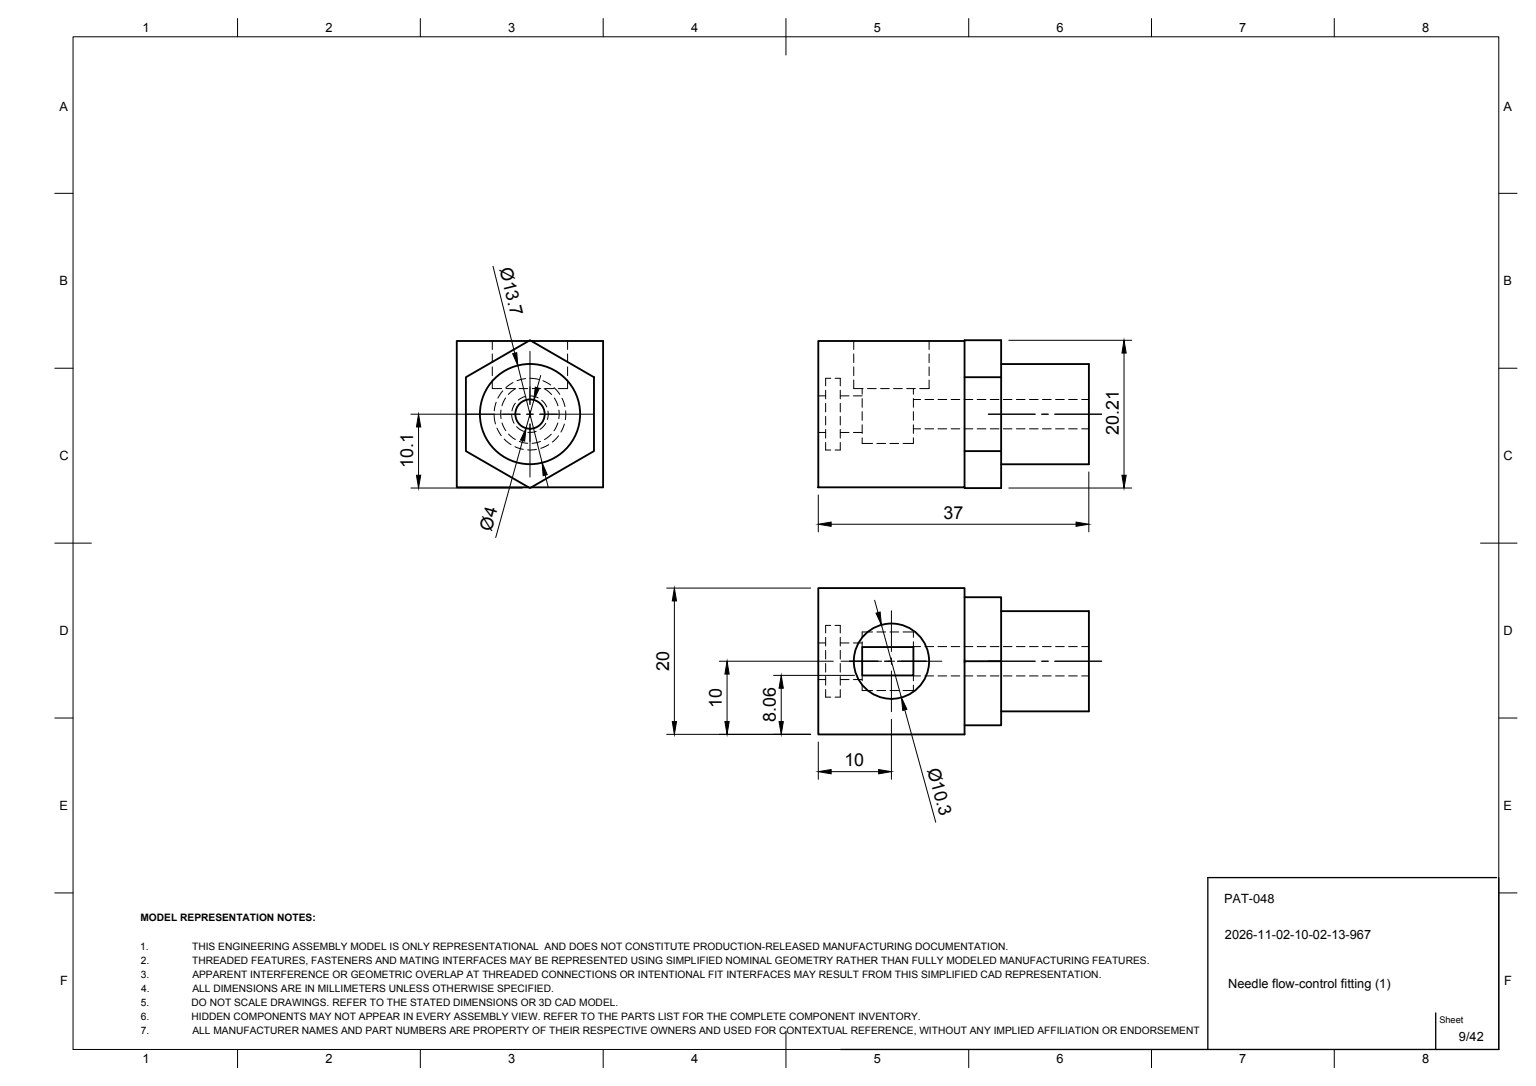
ISO-10303-21;
HEADER;
/* Generated by software containing ST-Developer
 * from STEP Tools, Inc. (www.steptools.com) 
 */

FILE_DESCRIPTION(
/* description */ ('Guided pneumatic stop gate'),
/* implementation_level */ '2;1');

FILE_NAME(
/* name */ 'Needle flow-control fitting (1).step',
/* time_stamp */ '2026-10-27T21:43:45-07:00',
/* author */ (''),
/* organization */ (''),
/* preprocessor_version */ 'ST-DEVELOPER v20.2',
/* originating_system */ 'Autodesk Translation Framework v15.17.0.0',
/* authorisation */ '');

FILE_SCHEMA (('AUTOMOTIVE_DESIGN { 1 0 10303 214 3 1 1 }'));
ENDSEC;

DATA;
#10=MECHANICAL_DESIGN_GEOMETRIC_PRESENTATION_REPRESENTATION('',(#539),#14392);
#455=SHAPE_REPRESENTATION_RELATIONSHIP('SRR','None',#14589,#497);
#497=ADVANCED_BREP_SHAPE_REPRESENTATION('',(#581),#14351);
#539=STYLED_ITEM('',(#14884),#581);
#581=MANIFOLD_SOLID_BREP('Body1',#7879);
#653=FACE_BOUND('',#1731,.T.);
#654=FACE_BOUND('',#1733,.T.);
#655=FACE_BOUND('',#1737,.T.);
#656=FACE_BOUND('',#1739,.T.);
#657=FACE_BOUND('',#1743,.T.);
#658=FACE_BOUND('',#1747,.T.);
#659=FACE_BOUND('',#1751,.T.);
#660=FACE_BOUND('',#1755,.T.);
#661=FACE_BOUND('',#1766,.T.);
#897=PLANE('',#8583);
#898=PLANE('',#8584);
#899=PLANE('',#8592);
#900=PLANE('',#8594);
#901=PLANE('',#8599);
#902=PLANE('',#8601);
#903=PLANE('',#8602);
#904=PLANE('',#8603);
#905=PLANE('',#8604);
#906=PLANE('',#8605);
#907=PLANE('',#8606);
#908=PLANE('',#8607);
#909=PLANE('',#8608);
#910=PLANE('',#8609);
#911=PLANE('',#8611);
#912=PLANE('',#8612);
#913=PLANE('',#8613);
#914=PLANE('',#8614);
#915=PLANE('',#8615);
#916=PLANE('',#8616);
#917=PLANE('',#8617);
#918=PLANE('',#8622);
#1216=FACE_OUTER_BOUND('',#1729,.T.);
#1217=FACE_OUTER_BOUND('',#1730,.T.);
#1218=FACE_OUTER_BOUND('',#1732,.T.);
#1219=FACE_OUTER_BOUND('',#1734,.T.);
#1220=FACE_OUTER_BOUND('',#1735,.T.);
#1221=FACE_OUTER_BOUND('',#1736,.T.);
#1222=FACE_OUTER_BOUND('',#1738,.T.);
#1223=FACE_OUTER_BOUND('',#1740,.T.);
#1224=FACE_OUTER_BOUND('',#1741,.T.);
#1225=FACE_OUTER_BOUND('',#1742,.T.);
#1226=FACE_OUTER_BOUND('',#1744,.T.);
#1227=FACE_OUTER_BOUND('',#1745,.T.);
#1228=FACE_OUTER_BOUND('',#1746,.T.);
#1229=FACE_OUTER_BOUND('',#1748,.T.);
#1230=FACE_OUTER_BOUND('',#1749,.T.);
#1231=FACE_OUTER_BOUND('',#1750,.T.);
#1232=FACE_OUTER_BOUND('',#1752,.T.);
#1233=FACE_OUTER_BOUND('',#1753,.T.);
#1234=FACE_OUTER_BOUND('',#1754,.T.);
#1235=FACE_OUTER_BOUND('',#1756,.T.);
#1236=FACE_OUTER_BOUND('',#1757,.T.);
#1237=FACE_OUTER_BOUND('',#1758,.T.);
#1238=FACE_OUTER_BOUND('',#1759,.T.);
#1239=FACE_OUTER_BOUND('',#1760,.T.);
#1240=FACE_OUTER_BOUND('',#1761,.T.);
#1241=FACE_OUTER_BOUND('',#1762,.T.);
#1242=FACE_OUTER_BOUND('',#1763,.T.);
#1243=FACE_OUTER_BOUND('',#1764,.T.);
#1244=FACE_OUTER_BOUND('',#1765,.T.);
#1729=EDGE_LOOP('',(#5720,#5721,#5722,#5723));
#1730=EDGE_LOOP('',(#5724));
#1731=EDGE_LOOP('',(#5725,#5726,#5727,#5728));
#1732=EDGE_LOOP('',(#5729,#5730));
#1733=EDGE_LOOP('',(#5731));
#1734=EDGE_LOOP('',(#5732,#5733,#5734,#5735));
#1735=EDGE_LOOP('',(#5736,#5737,#5738,#5739));
#1736=EDGE_LOOP('',(#5740));
#1737=EDGE_LOOP('',(#5741));
#1738=EDGE_LOOP('',(#5742));
#1739=EDGE_LOOP('',(#5743));
#1740=EDGE_LOOP('',(#5744,#5745,#5746,#5747));
#1741=EDGE_LOOP('',(#5748,#5749,#5750,#5751));
#1742=EDGE_LOOP('',(#5752,#5753));
#1743=EDGE_LOOP('',(#5754));
#1744=EDGE_LOOP('',(#5755,#5756,#5757,#5758,#5759,#5760));
#1745=EDGE_LOOP('',(#5761,#5762,#5763,#5764));
#1746=EDGE_LOOP('',(#5765,#5766,#5767,#5768,#5769,#5770));
#1747=EDGE_LOOP('',(#5771));
#1748=EDGE_LOOP('',(#5772,#5773,#5774,#5775));
#1749=EDGE_LOOP('',(#5776,#5777,#5778,#5779,#5780,#5781));
#1750=EDGE_LOOP('',(#5782,#5783,#5784,#5785));
#1751=EDGE_LOOP('',(#5786));
#1752=EDGE_LOOP('',(#5787,#5788,#5789,#5790,#5791,#5792));
#1753=EDGE_LOOP('',(#5793,#5794,#5795));
#1754=EDGE_LOOP('',(#5796,#5797,#5798,#5799,#5800,#5801));
#1755=EDGE_LOOP('',(#5802));
#1756=EDGE_LOOP('',(#5803,#5804,#5805,#5806));
#1757=EDGE_LOOP('',(#5807,#5808,#5809,#5810,#5811));
#1758=EDGE_LOOP('',(#5812,#5813,#5814,#5815,#5816));
#1759=EDGE_LOOP('',(#5817,#5818,#5819,#5820));
#1760=EDGE_LOOP('',(#5821,#5822,#5823,#5824,#5825));
#1761=EDGE_LOOP('',(#5826,#5827,#5828,#5829,#5830));
#1762=EDGE_LOOP('',(#5831,#5832,#5833));
#1763=EDGE_LOOP('',(#5834,#5835,#5836,#5837));
#1764=EDGE_LOOP('',(#5838,#5839,#5840,#5841));
#1765=EDGE_LOOP('',(#5842));
#1766=EDGE_LOOP('',(#5843));
#2389=LINE('',#12355,#2934);
#2390=LINE('',#12360,#2935);
#2391=LINE('',#12362,#2936);
#2392=LINE('',#12364,#2937);
#2393=LINE('',#12365,#2938);
#2394=LINE('',#12376,#2939);
#2395=LINE('',#12385,#2940);
#2396=LINE('',#12388,#2941);
#2397=LINE('',#12396,#2942);
#2398=LINE('',#12398,#2943);
#2399=LINE('',#12400,#2944);
#2400=LINE('',#12402,#2945);
#2401=LINE('',#12404,#2946);
#2402=LINE('',#12405,#2947);
#2403=LINE('',#12409,#2948);
#2404=LINE('',#12411,#2949);
#2405=LINE('',#12413,#2950);
#2406=LINE('',#12414,#2951);
#2407=LINE('',#12417,#2952);
#2408=LINE('',#12418,#2953);
#2409=LINE('',#12420,#2954);
#2410=LINE('',#12421,#2955);
#2411=LINE('',#12424,#2956);
#2412=LINE('',#12425,#2957);
#2413=LINE('',#12428,#2958);
#2414=LINE('',#12429,#2959);
#2415=LINE('',#12430,#2960);
#2416=LINE('',#12434,#2961);
#2417=LINE('',#12436,#2962);
#2418=LINE('',#12437,#2963);
#2419=LINE('',#12440,#2964);
#2420=LINE('',#12441,#2965);
#2421=LINE('',#12445,#2966);
#2422=LINE('',#12447,#2967);
#2423=LINE('',#12449,#2968);
#2424=LINE('',#12451,#2969);
#2425=LINE('',#12453,#2970);
#2426=LINE('',#12454,#2971);
#2427=LINE('',#12458,#2972);
#2428=LINE('',#12459,#2973);
#2429=LINE('',#12462,#2974);
#2430=LINE('',#12463,#2975);
#2431=LINE('',#12465,#2976);
#2432=LINE('',#12466,#2977);
#2433=LINE('',#12468,#2978);
#2434=LINE('',#12470,#2979);
#2435=LINE('',#12475,#2980);
#2436=LINE('',#12479,#2981);
#2934=VECTOR('',#9888,0.515);
#2935=VECTOR('',#9893,1.);
#2936=VECTOR('',#9894,1.);
#2937=VECTOR('',#9895,1.);
#2938=VECTOR('',#9896,1.);
#2939=VECTOR('',#9911,0.49);
#2940=VECTOR('',#9924,0.25);
#2941=VECTOR('',#9927,0.25);
#2942=VECTOR('',#9936,1.);
#2943=VECTOR('',#9937,1.);
#2944=VECTOR('',#9938,1.);
#2945=VECTOR('',#9939,1.);
#2946=VECTOR('',#9940,1.);
#2947=VECTOR('',#9941,1.);
#2948=VECTOR('',#9944,1.);
#2949=VECTOR('',#9945,1.);
#2950=VECTOR('',#9946,1.);
#2951=VECTOR('',#9947,1.);
#2952=VECTOR('',#9950,1.);
#2953=VECTOR('',#9951,1.);
#2954=VECTOR('',#9952,1.);
#2955=VECTOR('',#9953,1.);
#2956=VECTOR('',#9956,1.);
#2957=VECTOR('',#9957,1.);
#2958=VECTOR('',#9960,1.);
#2959=VECTOR('',#9961,1.);
#2960=VECTOR('',#9962,1.);
#2961=VECTOR('',#9967,1.);
#2962=VECTOR('',#9968,1.);
#2963=VECTOR('',#9969,1.);
#2964=VECTOR('',#9972,1.);
#2965=VECTOR('',#9973,1.);
#2966=VECTOR('',#9976,1.);
#2967=VECTOR('',#9977,1.);
#2968=VECTOR('',#9978,1.);
#2969=VECTOR('',#9979,1.);
#2970=VECTOR('',#9980,1.);
#2971=VECTOR('',#9981,1.);
#2972=VECTOR('',#9986,1.);
#2973=VECTOR('',#9987,1.);
#2974=VECTOR('',#9990,1.);
#2975=VECTOR('',#9991,1.);
#2976=VECTOR('',#9994,1.);
#2977=VECTOR('',#9995,1.);
#2978=VECTOR('',#9998,1.);
#2979=VECTOR('',#10001,1.);
#2980=VECTOR('',#10008,0.2);
#2981=VECTOR('',#10013,0.685);
#3445=CIRCLE('',#8581,0.515);
#3446=CIRCLE('',#8582,0.515);
#3447=CIRCLE('',#8585,0.4);
#3448=CIRCLE('',#8586,0.25);
#3449=CIRCLE('',#8588,0.4);
#3450=CIRCLE('',#8590,0.49);
#3451=CIRCLE('',#8591,0.49);
#3452=CIRCLE('',#8593,0.25);
#3453=CIRCLE('',#8595,0.25);
#3454=CIRCLE('',#8598,0.25);
#3455=CIRCLE('',#8600,0.2);
#3456=CIRCLE('',#8610,0.685);
#3457=CIRCLE('',#8619,0.2);
#3458=CIRCLE('',#8621,0.685);
#3861=VERTEX_POINT('',#12352);
#3862=VERTEX_POINT('',#12354);
#3863=VERTEX_POINT('',#12358);
#3864=VERTEX_POINT('',#12359);
#3865=VERTEX_POINT('',#12361);
#3866=VERTEX_POINT('',#12363);
#3867=VERTEX_POINT('',#12368);
#3868=VERTEX_POINT('',#12373);
#3869=VERTEX_POINT('',#12375);
#3870=VERTEX_POINT('',#12379);
#3871=VERTEX_POINT('',#12382);
#3872=VERTEX_POINT('',#12387);
#3873=VERTEX_POINT('',#12391);
#3874=VERTEX_POINT('',#12394);
#3875=VERTEX_POINT('',#12395);
#3876=VERTEX_POINT('',#12397);
#3877=VERTEX_POINT('',#12399);
#3878=VERTEX_POINT('',#12401);
#3879=VERTEX_POINT('',#12403);
#3880=VERTEX_POINT('',#12407);
#3881=VERTEX_POINT('',#12408);
#3882=VERTEX_POINT('',#12410);
#3883=VERTEX_POINT('',#12412);
#3884=VERTEX_POINT('',#12416);
#3885=VERTEX_POINT('',#12419);
#3886=VERTEX_POINT('',#12423);
#3887=VERTEX_POINT('',#12427);
#3888=VERTEX_POINT('',#12433);
#3889=VERTEX_POINT('',#12435);
#3890=VERTEX_POINT('',#12439);
#3891=VERTEX_POINT('',#12443);
#3892=VERTEX_POINT('',#12444);
#3893=VERTEX_POINT('',#12446);
#3894=VERTEX_POINT('',#12448);
#3895=VERTEX_POINT('',#12450);
#3896=VERTEX_POINT('',#12452);
#3897=VERTEX_POINT('',#12455);
#3898=VERTEX_POINT('',#12461);
#3899=VERTEX_POINT('',#12474);
#3900=VERTEX_POINT('',#12478);
#4558=EDGE_CURVE('',#3861,#3861,#3445,.T.);
#4559=EDGE_CURVE('',#3861,#3862,#2389,.T.);
#4560=EDGE_CURVE('',#3862,#3862,#3446,.T.);
#4561=EDGE_CURVE('',#3863,#3864,#2390,.T.);
#4562=EDGE_CURVE('',#3865,#3863,#2391,.T.);
#4563=EDGE_CURVE('',#3866,#3865,#2392,.T.);
#4564=EDGE_CURVE('',#3864,#3866,#2393,.T.);
#4565=EDGE_CURVE('',#3865,#3863,#3447,.T.);
#4566=EDGE_CURVE('',#3867,#3867,#3448,.T.);
#4567=EDGE_CURVE('',#3866,#3864,#3449,.T.);
#4568=EDGE_CURVE('',#3868,#3868,#3450,.T.);
#4569=EDGE_CURVE('',#3868,#3869,#2394,.T.);
#4570=EDGE_CURVE('',#3869,#3869,#3451,.T.);
#4571=EDGE_CURVE('',#3870,#3870,#3452,.T.);
#4572=EDGE_CURVE('',#3871,#3871,#3453,.T.);
#4573=EDGE_CURVE('',#3867,#3871,#2395,.T.);
#4574=EDGE_CURVE('',#3870,#3872,#2396,.T.);
#4575=EDGE_CURVE('',#3872,#3872,#3454,.T.);
#4576=EDGE_CURVE('',#3873,#3873,#3455,.T.);
#4577=EDGE_CURVE('',#3874,#3875,#2397,.T.);
#4578=EDGE_CURVE('',#3875,#3876,#2398,.T.);
#4579=EDGE_CURVE('',#3876,#3877,#2399,.T.);
#4580=EDGE_CURVE('',#3878,#3877,#2400,.T.);
#4581=EDGE_CURVE('',#3879,#3878,#2401,.T.);
#4582=EDGE_CURVE('',#3874,#3879,#2402,.T.);
#4583=EDGE_CURVE('',#3880,#3881,#2403,.T.);
#4584=EDGE_CURVE('',#3881,#3882,#2404,.T.);
#4585=EDGE_CURVE('',#3883,#3882,#2405,.T.);
#4586=EDGE_CURVE('',#3880,#3883,#2406,.T.);
#4587=EDGE_CURVE('',#3884,#3877,#2407,.T.);
#4588=EDGE_CURVE('',#3884,#3880,#2408,.T.);
#4589=EDGE_CURVE('',#3885,#3883,#2409,.T.);
#4590=EDGE_CURVE('',#3878,#3885,#2410,.T.);
#4591=EDGE_CURVE('',#3886,#3885,#2411,.T.);
#4592=EDGE_CURVE('',#3879,#3886,#2412,.T.);
#4593=EDGE_CURVE('',#3881,#3887,#2413,.T.);
#4594=EDGE_CURVE('',#3874,#3887,#2414,.T.);
#4595=EDGE_CURVE('',#3882,#3886,#2415,.T.);
#4596=EDGE_CURVE('',#3888,#3887,#2416,.T.);
#4597=EDGE_CURVE('',#3884,#3889,#2417,.T.);
#4598=EDGE_CURVE('',#3889,#3888,#2418,.T.);
#4599=EDGE_CURVE('',#3877,#3890,#2419,.T.);
#4600=EDGE_CURVE('',#3890,#3884,#2420,.T.);
#4601=EDGE_CURVE('',#3891,#3892,#2421,.T.);
#4602=EDGE_CURVE('',#3893,#3891,#2422,.T.);
#4603=EDGE_CURVE('',#3894,#3893,#2423,.T.);
#4604=EDGE_CURVE('',#3895,#3894,#2424,.T.);
#4605=EDGE_CURVE('',#3896,#3895,#2425,.T.);
#4606=EDGE_CURVE('',#3892,#3896,#2426,.T.);
#4607=EDGE_CURVE('',#3897,#3897,#3456,.T.);
#4608=EDGE_CURVE('',#3891,#3876,#2427,.T.);
#4609=EDGE_CURVE('',#3893,#3875,#2428,.T.);
#4610=EDGE_CURVE('',#3898,#3874,#2429,.T.);
#4611=EDGE_CURVE('',#3894,#3898,#2430,.T.);
#4612=EDGE_CURVE('',#3887,#3898,#2431,.T.);
#4613=EDGE_CURVE('',#3895,#3888,#2432,.T.);
#4614=EDGE_CURVE('',#3896,#3889,#2433,.T.);
#4615=EDGE_CURVE('',#3892,#3890,#2434,.T.);
#4616=EDGE_CURVE('',#3873,#3899,#2435,.T.);
#4617=EDGE_CURVE('',#3899,#3899,#3457,.T.);
#4618=EDGE_CURVE('',#3897,#3900,#2436,.T.);
#4619=EDGE_CURVE('',#3900,#3900,#3458,.T.);
#5720=ORIENTED_EDGE('',*,*,#4558,.F.);
#5721=ORIENTED_EDGE('',*,*,#4559,.T.);
#5722=ORIENTED_EDGE('',*,*,#4560,.F.);
#5723=ORIENTED_EDGE('',*,*,#4559,.F.);
#5724=ORIENTED_EDGE('',*,*,#4558,.T.);
#5725=ORIENTED_EDGE('',*,*,#4561,.F.);
#5726=ORIENTED_EDGE('',*,*,#4562,.F.);
#5727=ORIENTED_EDGE('',*,*,#4563,.F.);
#5728=ORIENTED_EDGE('',*,*,#4564,.F.);
#5729=ORIENTED_EDGE('',*,*,#4562,.T.);
#5730=ORIENTED_EDGE('',*,*,#4565,.F.);
#5731=ORIENTED_EDGE('',*,*,#4566,.T.);
#5732=ORIENTED_EDGE('',*,*,#4563,.T.);
#5733=ORIENTED_EDGE('',*,*,#4565,.T.);
#5734=ORIENTED_EDGE('',*,*,#4561,.T.);
#5735=ORIENTED_EDGE('',*,*,#4567,.F.);
#5736=ORIENTED_EDGE('',*,*,#4568,.F.);
#5737=ORIENTED_EDGE('',*,*,#4569,.T.);
#5738=ORIENTED_EDGE('',*,*,#4570,.T.);
#5739=ORIENTED_EDGE('',*,*,#4569,.F.);
#5740=ORIENTED_EDGE('',*,*,#4570,.F.);
#5741=ORIENTED_EDGE('',*,*,#4571,.F.);
#5742=ORIENTED_EDGE('',*,*,#4568,.T.);
#5743=ORIENTED_EDGE('',*,*,#4572,.F.);
#5744=ORIENTED_EDGE('',*,*,#4566,.F.);
#5745=ORIENTED_EDGE('',*,*,#4573,.T.);
#5746=ORIENTED_EDGE('',*,*,#4572,.T.);
#5747=ORIENTED_EDGE('',*,*,#4573,.F.);
#5748=ORIENTED_EDGE('',*,*,#4571,.T.);
#5749=ORIENTED_EDGE('',*,*,#4574,.T.);
#5750=ORIENTED_EDGE('',*,*,#4575,.F.);
#5751=ORIENTED_EDGE('',*,*,#4574,.F.);
#5752=ORIENTED_EDGE('',*,*,#4564,.T.);
#5753=ORIENTED_EDGE('',*,*,#4567,.T.);
#5754=ORIENTED_EDGE('',*,*,#4576,.F.);
#5755=ORIENTED_EDGE('',*,*,#4577,.T.);
#5756=ORIENTED_EDGE('',*,*,#4578,.T.);
#5757=ORIENTED_EDGE('',*,*,#4579,.T.);
#5758=ORIENTED_EDGE('',*,*,#4580,.F.);
#5759=ORIENTED_EDGE('',*,*,#4581,.F.);
#5760=ORIENTED_EDGE('',*,*,#4582,.F.);
#5761=ORIENTED_EDGE('',*,*,#4583,.T.);
#5762=ORIENTED_EDGE('',*,*,#4584,.T.);
#5763=ORIENTED_EDGE('',*,*,#4585,.F.);
#5764=ORIENTED_EDGE('',*,*,#4586,.F.);
#5765=ORIENTED_EDGE('',*,*,#4580,.T.);
#5766=ORIENTED_EDGE('',*,*,#4587,.F.);
#5767=ORIENTED_EDGE('',*,*,#4588,.T.);
#5768=ORIENTED_EDGE('',*,*,#4586,.T.);
#5769=ORIENTED_EDGE('',*,*,#4589,.F.);
#5770=ORIENTED_EDGE('',*,*,#4590,.F.);
#5771=ORIENTED_EDGE('',*,*,#4560,.T.);
#5772=ORIENTED_EDGE('',*,*,#4581,.T.);
#5773=ORIENTED_EDGE('',*,*,#4590,.T.);
#5774=ORIENTED_EDGE('',*,*,#4591,.F.);
#5775=ORIENTED_EDGE('',*,*,#4592,.F.);
#5776=ORIENTED_EDGE('',*,*,#4593,.T.);
#5777=ORIENTED_EDGE('',*,*,#4594,.F.);
#5778=ORIENTED_EDGE('',*,*,#4582,.T.);
#5779=ORIENTED_EDGE('',*,*,#4592,.T.);
#5780=ORIENTED_EDGE('',*,*,#4595,.F.);
#5781=ORIENTED_EDGE('',*,*,#4584,.F.);
#5782=ORIENTED_EDGE('',*,*,#4595,.T.);
#5783=ORIENTED_EDGE('',*,*,#4591,.T.);
#5784=ORIENTED_EDGE('',*,*,#4589,.T.);
#5785=ORIENTED_EDGE('',*,*,#4585,.T.);
#5786=ORIENTED_EDGE('',*,*,#4575,.T.);
#5787=ORIENTED_EDGE('',*,*,#4596,.T.);
#5788=ORIENTED_EDGE('',*,*,#4593,.F.);
#5789=ORIENTED_EDGE('',*,*,#4583,.F.);
#5790=ORIENTED_EDGE('',*,*,#4588,.F.);
#5791=ORIENTED_EDGE('',*,*,#4597,.T.);
#5792=ORIENTED_EDGE('',*,*,#4598,.T.);
#5793=ORIENTED_EDGE('',*,*,#4587,.T.);
#5794=ORIENTED_EDGE('',*,*,#4599,.T.);
#5795=ORIENTED_EDGE('',*,*,#4600,.T.);
#5796=ORIENTED_EDGE('',*,*,#4601,.F.);
#5797=ORIENTED_EDGE('',*,*,#4602,.F.);
#5798=ORIENTED_EDGE('',*,*,#4603,.F.);
#5799=ORIENTED_EDGE('',*,*,#4604,.F.);
#5800=ORIENTED_EDGE('',*,*,#4605,.F.);
#5801=ORIENTED_EDGE('',*,*,#4606,.F.);
#5802=ORIENTED_EDGE('',*,*,#4607,.T.);
#5803=ORIENTED_EDGE('',*,*,#4602,.T.);
#5804=ORIENTED_EDGE('',*,*,#4608,.T.);
#5805=ORIENTED_EDGE('',*,*,#4578,.F.);
#5806=ORIENTED_EDGE('',*,*,#4609,.F.);
#5807=ORIENTED_EDGE('',*,*,#4603,.T.);
#5808=ORIENTED_EDGE('',*,*,#4609,.T.);
#5809=ORIENTED_EDGE('',*,*,#4577,.F.);
#5810=ORIENTED_EDGE('',*,*,#4610,.F.);
#5811=ORIENTED_EDGE('',*,*,#4611,.F.);
#5812=ORIENTED_EDGE('',*,*,#4604,.T.);
#5813=ORIENTED_EDGE('',*,*,#4611,.T.);
#5814=ORIENTED_EDGE('',*,*,#4612,.F.);
#5815=ORIENTED_EDGE('',*,*,#4596,.F.);
#5816=ORIENTED_EDGE('',*,*,#4613,.F.);
#5817=ORIENTED_EDGE('',*,*,#4605,.T.);
#5818=ORIENTED_EDGE('',*,*,#4613,.T.);
#5819=ORIENTED_EDGE('',*,*,#4598,.F.);
#5820=ORIENTED_EDGE('',*,*,#4614,.F.);
#5821=ORIENTED_EDGE('',*,*,#4606,.T.);
#5822=ORIENTED_EDGE('',*,*,#4614,.T.);
#5823=ORIENTED_EDGE('',*,*,#4597,.F.);
#5824=ORIENTED_EDGE('',*,*,#4600,.F.);
#5825=ORIENTED_EDGE('',*,*,#4615,.F.);
#5826=ORIENTED_EDGE('',*,*,#4601,.T.);
#5827=ORIENTED_EDGE('',*,*,#4615,.T.);
#5828=ORIENTED_EDGE('',*,*,#4599,.F.);
#5829=ORIENTED_EDGE('',*,*,#4579,.F.);
#5830=ORIENTED_EDGE('',*,*,#4608,.F.);
#5831=ORIENTED_EDGE('',*,*,#4594,.T.);
#5832=ORIENTED_EDGE('',*,*,#4612,.T.);
#5833=ORIENTED_EDGE('',*,*,#4610,.T.);
#5834=ORIENTED_EDGE('',*,*,#4576,.T.);
#5835=ORIENTED_EDGE('',*,*,#4616,.T.);
#5836=ORIENTED_EDGE('',*,*,#4617,.T.);
#5837=ORIENTED_EDGE('',*,*,#4616,.F.);
#5838=ORIENTED_EDGE('',*,*,#4607,.F.);
#5839=ORIENTED_EDGE('',*,*,#4618,.T.);
#5840=ORIENTED_EDGE('',*,*,#4619,.T.);
#5841=ORIENTED_EDGE('',*,*,#4618,.F.);
#5842=ORIENTED_EDGE('',*,*,#4619,.F.);
#5843=ORIENTED_EDGE('',*,*,#4617,.F.);
#7274=CYLINDRICAL_SURFACE('',#8580,0.515);
#7275=CYLINDRICAL_SURFACE('',#8587,0.4);
#7276=CYLINDRICAL_SURFACE('',#8589,0.49);
#7277=CYLINDRICAL_SURFACE('',#8596,0.25);
#7278=CYLINDRICAL_SURFACE('',#8597,0.25);
#7279=CYLINDRICAL_SURFACE('',#8618,0.2);
#7280=CYLINDRICAL_SURFACE('',#8620,0.685);
#7498=ADVANCED_FACE('',(#1216),#7274,.F.);
#7499=ADVANCED_FACE('',(#1217,#653),#897,.T.);
#7500=ADVANCED_FACE('',(#1218,#654),#898,.F.);
#7501=ADVANCED_FACE('',(#1219),#7275,.F.);
#7502=ADVANCED_FACE('',(#1220),#7276,.F.);
#7503=ADVANCED_FACE('',(#1221,#655),#899,.F.);
#7504=ADVANCED_FACE('',(#1222,#656),#900,.T.);
#7505=ADVANCED_FACE('',(#1223),#7277,.F.);
#7506=ADVANCED_FACE('',(#1224),#7278,.F.);
#7507=ADVANCED_FACE('',(#1225,#657),#901,.T.);
#7508=ADVANCED_FACE('',(#1226),#902,.F.);
#7509=ADVANCED_FACE('',(#1227),#903,.T.);
#7510=ADVANCED_FACE('',(#1228,#658),#904,.T.);
#7511=ADVANCED_FACE('',(#1229),#905,.T.);
#7512=ADVANCED_FACE('',(#1230),#906,.T.);
#7513=ADVANCED_FACE('',(#1231,#659),#907,.T.);
#7514=ADVANCED_FACE('',(#1232),#908,.F.);
#7515=ADVANCED_FACE('',(#1233),#909,.T.);
#7516=ADVANCED_FACE('',(#1234,#660),#910,.F.);
#7517=ADVANCED_FACE('',(#1235),#911,.T.);
#7518=ADVANCED_FACE('',(#1236),#912,.T.);
#7519=ADVANCED_FACE('',(#1237),#913,.T.);
#7520=ADVANCED_FACE('',(#1238),#914,.T.);
#7521=ADVANCED_FACE('',(#1239),#915,.T.);
#7522=ADVANCED_FACE('',(#1240),#916,.T.);
#7523=ADVANCED_FACE('',(#1241),#917,.T.);
#7524=ADVANCED_FACE('',(#1242),#7279,.F.);
#7525=ADVANCED_FACE('',(#1243),#7280,.T.);
#7526=ADVANCED_FACE('',(#1244,#661),#918,.F.);
#7879=CLOSED_SHELL('',(#7498,#7499,#7500,#7501,#7502,#7503,#7504,#7505,
#7506,#7507,#7508,#7509,#7510,#7511,#7512,#7513,#7514,#7515,#7516,#7517,
#7518,#7519,#7520,#7521,#7522,#7523,#7524,#7525,#7526));
#8579=AXIS2_PLACEMENT_3D('',#12350,#9882,#9883);
#8580=AXIS2_PLACEMENT_3D('',#12351,#9884,#9885);
#8581=AXIS2_PLACEMENT_3D('',#12353,#9886,#9887);
#8582=AXIS2_PLACEMENT_3D('',#12356,#9889,#9890);
#8583=AXIS2_PLACEMENT_3D('',#12357,#9891,#9892);
#8584=AXIS2_PLACEMENT_3D('',#12366,#9897,#9898);
#8585=AXIS2_PLACEMENT_3D('',#12367,#9899,#9900);
#8586=AXIS2_PLACEMENT_3D('',#12369,#9901,#9902);
#8587=AXIS2_PLACEMENT_3D('',#12370,#9903,#9904);
#8588=AXIS2_PLACEMENT_3D('',#12371,#9905,#9906);
#8589=AXIS2_PLACEMENT_3D('',#12372,#9907,#9908);
#8590=AXIS2_PLACEMENT_3D('',#12374,#9909,#9910);
#8591=AXIS2_PLACEMENT_3D('',#12377,#9912,#9913);
#8592=AXIS2_PLACEMENT_3D('',#12378,#9914,#9915);
#8593=AXIS2_PLACEMENT_3D('',#12380,#9916,#9917);
#8594=AXIS2_PLACEMENT_3D('',#12381,#9918,#9919);
#8595=AXIS2_PLACEMENT_3D('',#12383,#9920,#9921);
#8596=AXIS2_PLACEMENT_3D('',#12384,#9922,#9923);
#8597=AXIS2_PLACEMENT_3D('',#12386,#9925,#9926);
#8598=AXIS2_PLACEMENT_3D('',#12389,#9928,#9929);
#8599=AXIS2_PLACEMENT_3D('',#12390,#9930,#9931);
#8600=AXIS2_PLACEMENT_3D('',#12392,#9932,#9933);
#8601=AXIS2_PLACEMENT_3D('',#12393,#9934,#9935);
#8602=AXIS2_PLACEMENT_3D('',#12406,#9942,#9943);
#8603=AXIS2_PLACEMENT_3D('',#12415,#9948,#9949);
#8604=AXIS2_PLACEMENT_3D('',#12422,#9954,#9955);
#8605=AXIS2_PLACEMENT_3D('',#12426,#9958,#9959);
#8606=AXIS2_PLACEMENT_3D('',#12431,#9963,#9964);
#8607=AXIS2_PLACEMENT_3D('',#12432,#9965,#9966);
#8608=AXIS2_PLACEMENT_3D('',#12438,#9970,#9971);
#8609=AXIS2_PLACEMENT_3D('',#12442,#9974,#9975);
#8610=AXIS2_PLACEMENT_3D('',#12456,#9982,#9983);
#8611=AXIS2_PLACEMENT_3D('',#12457,#9984,#9985);
#8612=AXIS2_PLACEMENT_3D('',#12460,#9988,#9989);
#8613=AXIS2_PLACEMENT_3D('',#12464,#9992,#9993);
#8614=AXIS2_PLACEMENT_3D('',#12467,#9996,#9997);
#8615=AXIS2_PLACEMENT_3D('',#12469,#9999,#10000);
#8616=AXIS2_PLACEMENT_3D('',#12471,#10002,#10003);
#8617=AXIS2_PLACEMENT_3D('',#12472,#10004,#10005);
#8618=AXIS2_PLACEMENT_3D('',#12473,#10006,#10007);
#8619=AXIS2_PLACEMENT_3D('',#12476,#10009,#10010);
#8620=AXIS2_PLACEMENT_3D('',#12477,#10011,#10012);
#8621=AXIS2_PLACEMENT_3D('',#12480,#10014,#10015);
#8622=AXIS2_PLACEMENT_3D('',#12481,#10016,#10017);
#9882=DIRECTION('axis',(0.,0.,1.));
#9883=DIRECTION('refdir',(1.,0.,0.));
#9884=DIRECTION('center_axis',(1.,0.,0.));
#9885=DIRECTION('ref_axis',(0.,0.,-1.));
#9886=DIRECTION('center_axis',(1.,0.,0.));
#9887=DIRECTION('ref_axis',(0.,0.,-1.));
#9888=DIRECTION('',(1.,0.,0.));
#9889=DIRECTION('center_axis',(-1.,0.,0.));
#9890=DIRECTION('ref_axis',(0.,0.,-1.));
#9891=DIRECTION('center_axis',(1.,0.,0.));
#9892=DIRECTION('ref_axis',(0.,0.,-1.));
#9893=DIRECTION('',(0.,0.,-1.));
#9894=DIRECTION('',(0.,-1.,0.));
#9895=DIRECTION('',(0.,0.,1.));
#9896=DIRECTION('',(0.,1.,0.));
#9897=DIRECTION('center_axis',(0.,0.,1.));
#9898=DIRECTION('ref_axis',(1.,0.,0.));
#9899=DIRECTION('center_axis',(0.,0.,1.));
#9900=DIRECTION('ref_axis',(1.,0.,0.));
#9901=DIRECTION('center_axis',(0.,0.,1.));
#9902=DIRECTION('ref_axis',(1.,0.,0.));
#9903=DIRECTION('center_axis',(0.,0.,1.));
#9904=DIRECTION('ref_axis',(-1.,1.22464679914735E-16,0.));
#9905=DIRECTION('center_axis',(0.,0.,1.));
#9906=DIRECTION('ref_axis',(1.,0.,0.));
#9907=DIRECTION('center_axis',(0.,0.,1.));
#9908=DIRECTION('ref_axis',(1.,0.,0.));
#9909=DIRECTION('center_axis',(0.,0.,1.));
#9910=DIRECTION('ref_axis',(1.,0.,0.));
#9911=DIRECTION('',(0.,0.,1.));
#9912=DIRECTION('center_axis',(0.,0.,1.));
#9913=DIRECTION('ref_axis',(1.,0.,0.));
#9914=DIRECTION('center_axis',(0.,0.,1.));
#9915=DIRECTION('ref_axis',(1.,0.,0.));
#9916=DIRECTION('center_axis',(0.,0.,-1.));
#9917=DIRECTION('ref_axis',(1.,0.,0.));
#9918=DIRECTION('center_axis',(0.,0.,1.));
#9919=DIRECTION('ref_axis',(1.,0.,0.));
#9920=DIRECTION('center_axis',(0.,0.,1.));
#9921=DIRECTION('ref_axis',(1.,0.,0.));
#9922=DIRECTION('center_axis',(0.,0.,1.));
#9923=DIRECTION('ref_axis',(1.,0.,0.));
#9924=DIRECTION('',(0.,0.,1.));
#9925=DIRECTION('center_axis',(0.,0.,1.));
#9926=DIRECTION('ref_axis',(1.,0.,0.));
#9927=DIRECTION('',(0.,0.,1.));
#9928=DIRECTION('center_axis',(0.,0.,-1.));
#9929=DIRECTION('ref_axis',(1.,0.,0.));
#9930=DIRECTION('center_axis',(0.,0.,1.));
#9931=DIRECTION('ref_axis',(1.,0.,0.));
#9932=DIRECTION('center_axis',(0.,0.,1.));
#9933=DIRECTION('ref_axis',(1.,0.,0.));
#9934=DIRECTION('center_axis',(0.,0.,1.));
#9935=DIRECTION('ref_axis',(1.,0.,0.));
#9936=DIRECTION('',(0.5,-0.866025403784439,0.));
#9937=DIRECTION('',(1.,0.,0.));
#9938=DIRECTION('',(0.5,0.866025403784439,0.));
#9939=DIRECTION('',(0.,1.,0.));
#9940=DIRECTION('',(1.,0.,0.));
#9941=DIRECTION('',(0.,-1.,0.));
#9942=DIRECTION('center_axis',(0.,1.,0.));
#9943=DIRECTION('ref_axis',(-1.,0.,0.));
#9944=DIRECTION('',(-1.,0.,0.));
#9945=DIRECTION('',(0.,0.,1.));
#9946=DIRECTION('',(-1.,0.,0.));
#9947=DIRECTION('',(0.,0.,1.));
#9948=DIRECTION('center_axis',(1.,0.,0.));
#9949=DIRECTION('ref_axis',(0.,1.,0.));
#9950=DIRECTION('',(0.,-1.,0.));
#9951=DIRECTION('',(0.,1.,0.));
#9952=DIRECTION('',(0.,1.,0.));
#9953=DIRECTION('',(0.,0.,1.));
#9954=DIRECTION('center_axis',(0.,-1.,0.));
#9955=DIRECTION('ref_axis',(1.,0.,0.));
#9956=DIRECTION('',(1.,0.,0.));
#9957=DIRECTION('',(0.,0.,1.));
#9958=DIRECTION('center_axis',(-1.,0.,0.));
#9959=DIRECTION('ref_axis',(0.,-1.,0.));
#9960=DIRECTION('',(0.,-1.,0.));
#9961=DIRECTION('',(0.,1.,0.));
#9962=DIRECTION('',(0.,-1.,0.));
#9963=DIRECTION('center_axis',(0.,0.,1.));
#9964=DIRECTION('ref_axis',(1.,0.,0.));
#9965=DIRECTION('center_axis',(0.,0.,1.));
#9966=DIRECTION('ref_axis',(1.,0.,0.));
#9967=DIRECTION('',(-0.5,-0.866025403784439,0.));
#9968=DIRECTION('',(-0.5,0.866025403784439,0.));
#9969=DIRECTION('',(-1.,0.,0.));
#9970=DIRECTION('center_axis',(0.,0.,1.));
#9971=DIRECTION('ref_axis',(1.,0.,0.));
#9972=DIRECTION('',(0.5,0.866025403784439,0.));
#9973=DIRECTION('',(-0.5,0.866025403784439,0.));
#9974=DIRECTION('center_axis',(0.,0.,1.));
#9975=DIRECTION('ref_axis',(1.,0.,0.));
#9976=DIRECTION('',(0.5,0.866025403784439,0.));
#9977=DIRECTION('',(1.,0.,0.));
#9978=DIRECTION('',(0.5,-0.866025403784439,0.));
#9979=DIRECTION('',(-0.5,-0.866025403784439,0.));
#9980=DIRECTION('',(-1.,0.,0.));
#9981=DIRECTION('',(-0.5,0.866025403784439,0.));
#9982=DIRECTION('center_axis',(0.,0.,1.));
#9983=DIRECTION('ref_axis',(1.,0.,0.));
#9984=DIRECTION('center_axis',(0.,-1.,0.));
#9985=DIRECTION('ref_axis',(1.,0.,0.));
#9986=DIRECTION('',(0.,0.,1.));
#9987=DIRECTION('',(0.,0.,1.));
#9988=DIRECTION('center_axis',(-0.866025403784439,-0.5,0.));
#9989=DIRECTION('ref_axis',(0.5,-0.866025403784439,0.));
#9990=DIRECTION('',(0.5,-0.866025403784439,0.));
#9991=DIRECTION('',(0.,0.,1.));
#9992=DIRECTION('center_axis',(-0.866025403784439,0.5,0.));
#9993=DIRECTION('ref_axis',(-0.5,-0.866025403784439,0.));
#9994=DIRECTION('',(-0.5,-0.866025403784439,0.));
#9995=DIRECTION('',(0.,0.,1.));
#9996=DIRECTION('center_axis',(0.,1.,0.));
#9997=DIRECTION('ref_axis',(-1.,0.,0.));
#9998=DIRECTION('',(0.,0.,1.));
#9999=DIRECTION('center_axis',(0.866025403784439,0.5,0.));
#10000=DIRECTION('ref_axis',(-0.5,0.866025403784439,0.));
#10001=DIRECTION('',(0.,0.,1.));
#10002=DIRECTION('center_axis',(0.866025403784439,-0.5,0.));
#10003=DIRECTION('ref_axis',(0.5,0.866025403784439,0.));
#10004=DIRECTION('center_axis',(0.,0.,1.));
#10005=DIRECTION('ref_axis',(1.,0.,0.));
#10006=DIRECTION('center_axis',(0.,0.,1.));
#10007=DIRECTION('ref_axis',(1.,0.,0.));
#10008=DIRECTION('',(0.,0.,-1.));
#10009=DIRECTION('center_axis',(0.,0.,-1.));
#10010=DIRECTION('ref_axis',(1.,0.,0.));
#10011=DIRECTION('center_axis',(0.,0.,1.));
#10012=DIRECTION('ref_axis',(1.,0.,0.));
#10013=DIRECTION('',(0.,0.,-1.));
#10014=DIRECTION('center_axis',(0.,0.,1.));
#10015=DIRECTION('ref_axis',(1.,0.,0.));
#10016=DIRECTION('center_axis',(0.,0.,1.));
#10017=DIRECTION('ref_axis',(1.,0.,0.));
#12350=CARTESIAN_POINT('',(0.,0.,0.));
#12351=CARTESIAN_POINT('Origin',(0.35,11.8,8.5));
#12352=CARTESIAN_POINT('',(0.35,11.8,9.015));
#12353=CARTESIAN_POINT('Origin',(0.35,11.8,8.5));
#12354=CARTESIAN_POINT('',(1.,11.8,9.015));
#12355=CARTESIAN_POINT('',(0.35,11.8,9.015));
#12356=CARTESIAN_POINT('Origin',(1.,11.8,8.5));
#12357=CARTESIAN_POINT('Origin',(0.35,11.8,8.5));
#12358=CARTESIAN_POINT('',(0.35,11.6063508326896,8.9));
#12359=CARTESIAN_POINT('',(0.35,11.6063508326896,8.2));
#12360=CARTESIAN_POINT('',(0.35,11.6063508326896,8.2));
#12361=CARTESIAN_POINT('',(0.35,11.9936491673104,8.9));
#12362=CARTESIAN_POINT('',(0.35,11.8,8.9));
#12363=CARTESIAN_POINT('',(0.35,11.9936491673104,8.2));
#12364=CARTESIAN_POINT('',(0.35,11.9936491673104,8.2));
#12365=CARTESIAN_POINT('',(0.35,11.8,8.2));
#12366=CARTESIAN_POINT('Origin',(0.,11.8,8.9));
#12367=CARTESIAN_POINT('Origin',(0.,11.8,8.9));
#12368=CARTESIAN_POINT('',(-0.25,11.8,8.9));
#12369=CARTESIAN_POINT('Origin',(0.,11.8,8.9));
#12370=CARTESIAN_POINT('Origin',(0.,11.8,8.2));
#12371=CARTESIAN_POINT('Origin',(0.,11.8,8.2));
#12372=CARTESIAN_POINT('Origin',(0.,11.8,9.2));
#12373=CARTESIAN_POINT('',(-0.49,11.8,9.2));
#12374=CARTESIAN_POINT('Origin',(0.,11.8,9.2));
#12375=CARTESIAN_POINT('',(-0.49,11.8,9.4));
#12376=CARTESIAN_POINT('',(-0.49,11.8,9.2));
#12377=CARTESIAN_POINT('Origin',(0.,11.8,9.4));
#12378=CARTESIAN_POINT('Origin',(0.,11.8,9.4));
#12379=CARTESIAN_POINT('',(-0.25,11.8,9.4));
#12380=CARTESIAN_POINT('Origin',(0.,11.8,9.4));
#12381=CARTESIAN_POINT('Origin',(0.,11.8,9.2));
#12382=CARTESIAN_POINT('',(-0.25,11.8,9.2));
#12383=CARTESIAN_POINT('Origin',(0.,11.8,9.2));
#12384=CARTESIAN_POINT('Origin',(0.,11.8,8.8));
#12385=CARTESIAN_POINT('',(-0.25,11.8,8.8));
#12386=CARTESIAN_POINT('Origin',(0.,11.8,8.8));
#12387=CARTESIAN_POINT('',(-0.25,11.8,9.5));
#12388=CARTESIAN_POINT('',(-0.25,11.8,8.8));
#12389=CARTESIAN_POINT('Origin',(0.,11.8,9.5));
#12390=CARTESIAN_POINT('Origin',(0.,11.8,8.2));
#12391=CARTESIAN_POINT('',(-0.2,11.8,8.2));
#12392=CARTESIAN_POINT('Origin',(0.,11.8,8.2));
#12393=CARTESIAN_POINT('Origin',(0.,11.8,7.5));
#12394=CARTESIAN_POINT('',(-1.,11.7820508075689,7.5));
#12395=CARTESIAN_POINT('',(-0.505181485540923,10.925,7.5));
#12396=CARTESIAN_POINT('',(-1.01036297108185,11.8,7.5));
#12397=CARTESIAN_POINT('',(0.505181485540923,10.925,7.5));
#12398=CARTESIAN_POINT('',(-0.505181485540923,10.925,7.5));
#12399=CARTESIAN_POINT('',(1.,11.7820508075689,7.5));
#12400=CARTESIAN_POINT('',(0.505181485540923,10.925,7.5));
#12401=CARTESIAN_POINT('',(1.,10.8,7.5));
#12402=CARTESIAN_POINT('',(1.,10.8,7.5));
#12403=CARTESIAN_POINT('',(-1.,10.8,7.5));
#12404=CARTESIAN_POINT('',(-1.,10.8,7.5));
#12405=CARTESIAN_POINT('',(-1.,12.8,7.5));
#12406=CARTESIAN_POINT('Origin',(1.,12.8,7.5));
#12407=CARTESIAN_POINT('',(1.,12.8,7.5));
#12408=CARTESIAN_POINT('',(-1.,12.8,7.5));
#12409=CARTESIAN_POINT('',(1.,12.8,7.5));
#12410=CARTESIAN_POINT('',(-1.,12.8,9.5));
#12411=CARTESIAN_POINT('',(-1.,12.8,7.5));
#12412=CARTESIAN_POINT('',(1.,12.8,9.5));
#12413=CARTESIAN_POINT('',(1.,12.8,9.5));
#12414=CARTESIAN_POINT('',(1.,12.8,7.5));
#12415=CARTESIAN_POINT('Origin',(1.,10.8,7.5));
#12416=CARTESIAN_POINT('',(1.,11.8179491924311,7.5));
#12417=CARTESIAN_POINT('',(1.,11.3,7.5));
#12418=CARTESIAN_POINT('',(1.,10.8,7.5));
#12419=CARTESIAN_POINT('',(1.,10.8,9.5));
#12420=CARTESIAN_POINT('',(1.,10.8,9.5));
#12421=CARTESIAN_POINT('',(1.,10.8,7.5));
#12422=CARTESIAN_POINT('Origin',(-1.,10.8,7.5));
#12423=CARTESIAN_POINT('',(-1.,10.8,9.5));
#12424=CARTESIAN_POINT('',(-1.,10.8,9.5));
#12425=CARTESIAN_POINT('',(-1.,10.8,7.5));
#12426=CARTESIAN_POINT('Origin',(-1.,12.8,7.5));
#12427=CARTESIAN_POINT('',(-1.,11.8179491924311,7.5));
#12428=CARTESIAN_POINT('',(-1.,12.8,7.5));
#12429=CARTESIAN_POINT('',(-1.,12.3,7.5));
#12430=CARTESIAN_POINT('',(-1.,12.8,9.5));
#12431=CARTESIAN_POINT('Origin',(0.,11.8,9.5));
#12432=CARTESIAN_POINT('Origin',(0.,11.8,7.5));
#12433=CARTESIAN_POINT('',(-0.505181485540922,12.675,7.5));
#12434=CARTESIAN_POINT('',(-0.505181485540922,12.675,7.5));
#12435=CARTESIAN_POINT('',(0.505181485540923,12.675,7.5));
#12436=CARTESIAN_POINT('',(1.01036297108185,11.8,7.5));
#12437=CARTESIAN_POINT('',(0.505181485540923,12.675,7.5));
#12438=CARTESIAN_POINT('Origin',(0.,11.8,7.5));
#12439=CARTESIAN_POINT('',(1.01036297108185,11.8,7.5));
#12440=CARTESIAN_POINT('',(0.505181485540923,10.925,7.5));
#12441=CARTESIAN_POINT('',(1.01036297108185,11.8,7.5));
#12442=CARTESIAN_POINT('Origin',(0.,11.8,7.));
#12443=CARTESIAN_POINT('',(0.505181485540923,10.925,7.));
#12444=CARTESIAN_POINT('',(1.01036297108185,11.8,7.));
#12445=CARTESIAN_POINT('',(0.505181485540923,10.925,7.));
#12446=CARTESIAN_POINT('',(-0.505181485540923,10.925,7.));
#12447=CARTESIAN_POINT('',(-0.505181485540923,10.925,7.));
#12448=CARTESIAN_POINT('',(-1.01036297108185,11.8,7.));
#12449=CARTESIAN_POINT('',(-1.01036297108185,11.8,7.));
#12450=CARTESIAN_POINT('',(-0.505181485540922,12.675,7.));
#12451=CARTESIAN_POINT('',(-0.505181485540922,12.675,7.));
#12452=CARTESIAN_POINT('',(0.505181485540923,12.675,7.));
#12453=CARTESIAN_POINT('',(0.505181485540923,12.675,7.));
#12454=CARTESIAN_POINT('',(1.01036297108185,11.8,7.));
#12455=CARTESIAN_POINT('',(-0.685,11.8,7.));
#12456=CARTESIAN_POINT('Origin',(0.,11.8,7.));
#12457=CARTESIAN_POINT('Origin',(-0.505181485540923,10.925,7.));
#12458=CARTESIAN_POINT('',(0.505181485540923,10.925,7.));
#12459=CARTESIAN_POINT('',(-0.505181485540923,10.925,7.));
#12460=CARTESIAN_POINT('Origin',(-1.01036297108185,11.8,7.));
#12461=CARTESIAN_POINT('',(-1.01036297108185,11.8,7.5));
#12462=CARTESIAN_POINT('',(-1.01036297108185,11.8,7.5));
#12463=CARTESIAN_POINT('',(-1.01036297108185,11.8,7.));
#12464=CARTESIAN_POINT('Origin',(-0.505181485540922,12.675,7.));
#12465=CARTESIAN_POINT('',(-0.505181485540922,12.675,7.5));
#12466=CARTESIAN_POINT('',(-0.505181485540922,12.675,7.));
#12467=CARTESIAN_POINT('Origin',(0.505181485540923,12.675,7.));
#12468=CARTESIAN_POINT('',(0.505181485540923,12.675,7.));
#12469=CARTESIAN_POINT('Origin',(1.01036297108185,11.8,7.));
#12470=CARTESIAN_POINT('',(1.01036297108185,11.8,7.));
#12471=CARTESIAN_POINT('Origin',(0.505181485540923,10.925,7.));
#12472=CARTESIAN_POINT('Origin',(0.,11.8,7.5));
#12473=CARTESIAN_POINT('Origin',(0.,11.8,5.8));
#12474=CARTESIAN_POINT('',(-0.2,11.8,5.8));
#12475=CARTESIAN_POINT('',(-0.2,11.8,5.8));
#12476=CARTESIAN_POINT('Origin',(0.,11.8,5.8));
#12477=CARTESIAN_POINT('Origin',(0.,11.8,5.8));
#12478=CARTESIAN_POINT('',(-0.685,11.8,5.8));
#12479=CARTESIAN_POINT('',(-0.685,11.8,5.8));
#12480=CARTESIAN_POINT('Origin',(0.,11.8,5.8));
#12481=CARTESIAN_POINT('Origin',(0.,11.8,5.8));
#14303=UNCERTAINTY_MEASURE_WITH_UNIT(LENGTH_MEASURE(0.001),#14393,
'DISTANCE_ACCURACY_VALUE',
'Maximum model space distance between geometric entities at asserted c
onnectivities');
#14344=UNCERTAINTY_MEASURE_WITH_UNIT(LENGTH_MEASURE(0.001),#14393,
'DISTANCE_ACCURACY_VALUE',
'Maximum model space distance between geometric entities at asserted c
onnectivities');
#14351=(
GEOMETRIC_REPRESENTATION_CONTEXT(3)
GLOBAL_UNCERTAINTY_ASSIGNED_CONTEXT((#14303))
GLOBAL_UNIT_ASSIGNED_CONTEXT((#14393,#14395,#14396))
REPRESENTATION_CONTEXT('','3D')
);
#14392=(
GEOMETRIC_REPRESENTATION_CONTEXT(3)
GLOBAL_UNCERTAINTY_ASSIGNED_CONTEXT((#14344))
GLOBAL_UNIT_ASSIGNED_CONTEXT((#14393,#14395,#14396))
REPRESENTATION_CONTEXT('','3D')
);
#14393=(
LENGTH_UNIT()
NAMED_UNIT(*)
SI_UNIT(.CENTI.,.METRE.)
);
#14395=(
NAMED_UNIT(*)
PLANE_ANGLE_UNIT()
SI_UNIT($,.RADIAN.)
);
#14396=(
NAMED_UNIT(*)
SI_UNIT($,.STERADIAN.)
SOLID_ANGLE_UNIT()
);
#14403=SHAPE_DEFINITION_REPRESENTATION(#14450,#14589);
#14450=PRODUCT_DEFINITION_SHAPE('',$,#14637);
#14589=SHAPE_REPRESENTATION('',(#8579),#14351);
#14630=PRODUCT_DEFINITION_CONTEXT('part definition',#14773,'design');
#14637=PRODUCT_DEFINITION('Needle flow-control fitting (1)',
'Needle flow-control fitting (1)',#14684,#14630);
#14684=PRODUCT_DEFINITION_FORMATION('',$,#14781);
#14773=APPLICATION_CONTEXT(
'Core Data for Automotive Mechanical Design Process');
#14774=PRODUCT_CONTEXT('part definition',#14773,'mechanical');
#14781=PRODUCT('Needle flow-control fitting (1)',
'Needle flow-control fitting (1)','Needle flow-control fitting (1)',(#14774));
#14878=COLOUR_RGB('Sky Blue',0.24,0.69,0.87);
#14879=FILL_AREA_STYLE_COLOUR('',#14878);
#14880=FILL_AREA_STYLE('',(#14879));
#14881=SURFACE_STYLE_FILL_AREA(#14880);
#14882=SURFACE_SIDE_STYLE('',(#14881));
#14883=SURFACE_STYLE_USAGE(.BOTH.,#14882);
#14884=PRESENTATION_STYLE_ASSIGNMENT((#14883));
ENDSEC;
END-ISO-10303-21;
